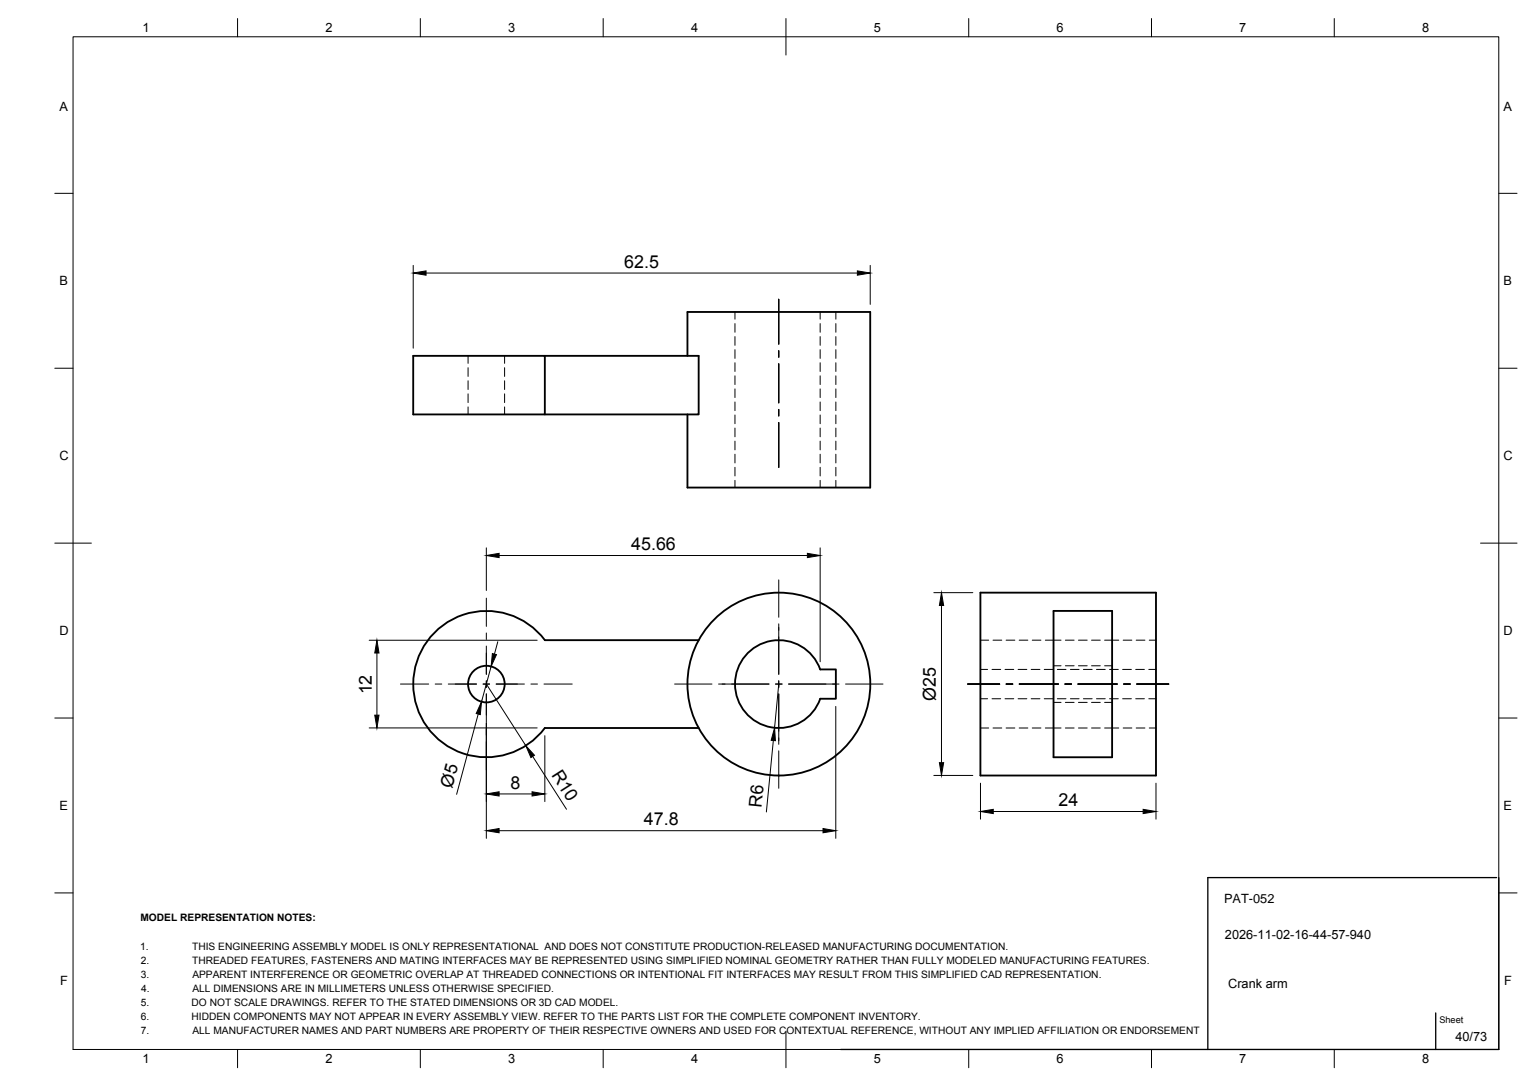
ISO-10303-21;
HEADER;
/* Generated by software containing ST-Developer
 * from STEP Tools, Inc. (www.steptools.com) 
 */

FILE_DESCRIPTION(
/* description */ ('Hand-crank gear train demonstrator'),
/* implementation_level */ '2;1');

FILE_NAME(
/* name */ 'Crank arm.step',
/* time_stamp */ '2026-10-28T03:22:13-07:00',
/* author */ (''),
/* organization */ (''),
/* preprocessor_version */ 'ST-DEVELOPER v20.2',
/* originating_system */ 'Autodesk Translation Framework v15.17.0.0',
/* authorisation */ '');

FILE_SCHEMA (('AUTOMOTIVE_DESIGN { 1 0 10303 214 3 1 1 }'));
ENDSEC;

DATA;
#10=MECHANICAL_DESIGN_GEOMETRIC_PRESENTATION_REPRESENTATION('',(#1236),#62758);
#1093=SHAPE_REPRESENTATION_RELATIONSHIP('SRR','None',#63068,#1157);
#1157=ADVANCED_BREP_SHAPE_REPRESENTATION('',(#1312),#62722);
#1236=STYLED_ITEM('',(#63455),#1312);
#1312=MANIFOLD_SOLID_BREP('Body1',#16419);
#1555=FACE_BOUND('',#3735,.T.);
#1556=FACE_BOUND('',#3739,.T.);
#1557=FACE_BOUND('',#3742,.T.);
#1558=FACE_BOUND('',#3745,.T.);
#1559=FACE_BOUND('',#3747,.T.);
#1906=PLANE('',#18042);
#1907=PLANE('',#18043);
#1908=PLANE('',#18044);
#1909=PLANE('',#18045);
#1910=PLANE('',#18053);
#1911=PLANE('',#18055);
#1912=PLANE('',#18056);
#1913=PLANE('',#18058);
#1914=PLANE('',#18061);
#2581=FACE_OUTER_BOUND('',#3730,.T.);
#2582=FACE_OUTER_BOUND('',#3731,.T.);
#2583=FACE_OUTER_BOUND('',#3732,.T.);
#2584=FACE_OUTER_BOUND('',#3733,.T.);
#2585=FACE_OUTER_BOUND('',#3734,.T.);
#2586=FACE_OUTER_BOUND('',#3736,.T.);
#2587=FACE_OUTER_BOUND('',#3737,.T.);
#2588=FACE_OUTER_BOUND('',#3738,.T.);
#2589=FACE_OUTER_BOUND('',#3740,.T.);
#2590=FACE_OUTER_BOUND('',#3741,.T.);
#2591=FACE_OUTER_BOUND('',#3743,.T.);
#2592=FACE_OUTER_BOUND('',#3744,.T.);
#2593=FACE_OUTER_BOUND('',#3746,.T.);
#3730=EDGE_LOOP('',(#12837,#12838,#12839,#12840));
#3731=EDGE_LOOP('',(#12841,#12842,#12843,#12844));
#3732=EDGE_LOOP('',(#12845,#12846,#12847,#12848));
#3733=EDGE_LOOP('',(#12849,#12850,#12851,#12852));
#3734=EDGE_LOOP('',(#12853));
#3735=EDGE_LOOP('',(#12854,#12855,#12856,#12857));
#3736=EDGE_LOOP('',(#12858,#12859,#12860,#12861));
#3737=EDGE_LOOP('',(#12862,#12863,#12864,#12865));
#3738=EDGE_LOOP('',(#12866,#12867,#12868,#12869));
#3739=EDGE_LOOP('',(#12870));
#3740=EDGE_LOOP('',(#12871,#12872,#12873,#12874));
#3741=EDGE_LOOP('',(#12875,#12876,#12877,#12878));
#3742=EDGE_LOOP('',(#12879));
#3743=EDGE_LOOP('',(#12880,#12881,#12882,#12883));
#3744=EDGE_LOOP('',(#12884,#12885,#12886,#12887));
#3745=EDGE_LOOP('',(#12888,#12889,#12890,#12891));
#3746=EDGE_LOOP('',(#12892));
#3747=EDGE_LOOP('',(#12893,#12894,#12895,#12896));
#4876=LINE('',#26186,#6008);
#4877=LINE('',#26191,#6009);
#4878=LINE('',#26193,#6010);
#4879=LINE('',#26195,#6011);
#4880=LINE('',#26196,#6012);
#4881=LINE('',#26199,#6013);
#4882=LINE('',#26201,#6014);
#4883=LINE('',#26202,#6015);
#4884=LINE('',#26205,#6016);
#4885=LINE('',#26207,#6017);
#4886=LINE('',#26208,#6018);
#4887=LINE('',#26218,#6019);
#4888=LINE('',#26222,#6020);
#4889=LINE('',#26226,#6021);
#4890=LINE('',#26229,#6022);
#4891=LINE('',#26232,#6023);
#4892=LINE('',#26233,#6024);
#4893=LINE('',#26236,#6025);
#4894=LINE('',#26239,#6026);
#4895=LINE('',#26242,#6027);
#6008=VECTOR('',#21187,0.25);
#6009=VECTOR('',#21192,1.);
#6010=VECTOR('',#21193,1.);
#6011=VECTOR('',#21194,1.);
#6012=VECTOR('',#21195,1.);
#6013=VECTOR('',#21198,1.);
#6014=VECTOR('',#21199,1.);
#6015=VECTOR('',#21200,1.);
#6016=VECTOR('',#21203,1.);
#6017=VECTOR('',#21204,1.);
#6018=VECTOR('',#21205,1.);
#6019=VECTOR('',#21218,1.);
#6020=VECTOR('',#21221,1.);
#6021=VECTOR('',#21226,1.);
#6022=VECTOR('',#21229,1.);
#6023=VECTOR('',#21232,1.);
#6024=VECTOR('',#21233,1.);
#6025=VECTOR('',#21236,1.);
#6026=VECTOR('',#21241,1.);
#6027=VECTOR('',#21244,1.25);
#6925=CIRCLE('',#18040,0.25);
#6926=CIRCLE('',#18041,0.25);
#6927=CIRCLE('',#18046,1.25);
#6928=CIRCLE('',#18047,0.6);
#6929=CIRCLE('',#18049,0.6);
#6930=CIRCLE('',#18051,1.);
#6931=CIRCLE('',#18052,1.);
#6932=CIRCLE('',#18054,1.25);
#6933=CIRCLE('',#18057,1.25);
#6934=CIRCLE('',#18060,1.25);
#7894=VERTEX_POINT('',#26183);
#7895=VERTEX_POINT('',#26185);
#7896=VERTEX_POINT('',#26189);
#7897=VERTEX_POINT('',#26190);
#7898=VERTEX_POINT('',#26192);
#7899=VERTEX_POINT('',#26194);
#7900=VERTEX_POINT('',#26198);
#7901=VERTEX_POINT('',#26200);
#7902=VERTEX_POINT('',#26204);
#7903=VERTEX_POINT('',#26206);
#7904=VERTEX_POINT('',#26210);
#7905=VERTEX_POINT('',#26216);
#7906=VERTEX_POINT('',#26217);
#7907=VERTEX_POINT('',#26219);
#7908=VERTEX_POINT('',#26221);
#7909=VERTEX_POINT('',#26225);
#7910=VERTEX_POINT('',#26227);
#7911=VERTEX_POINT('',#26231);
#7912=VERTEX_POINT('',#26235);
#7913=VERTEX_POINT('',#26241);
#9670=EDGE_CURVE('',#7894,#7894,#6925,.T.);
#9671=EDGE_CURVE('',#7894,#7895,#4876,.T.);
#9672=EDGE_CURVE('',#7895,#7895,#6926,.T.);
#9673=EDGE_CURVE('',#7896,#7897,#4877,.T.);
#9674=EDGE_CURVE('',#7896,#7898,#4878,.T.);
#9675=EDGE_CURVE('',#7899,#7898,#4879,.T.);
#9676=EDGE_CURVE('',#7897,#7899,#4880,.T.);
#9677=EDGE_CURVE('',#7900,#7896,#4881,.T.);
#9678=EDGE_CURVE('',#7900,#7901,#4882,.T.);
#9679=EDGE_CURVE('',#7898,#7901,#4883,.T.);
#9680=EDGE_CURVE('',#7902,#7900,#4884,.T.);
#9681=EDGE_CURVE('',#7903,#7902,#4885,.T.);
#9682=EDGE_CURVE('',#7901,#7903,#4886,.T.);
#9683=EDGE_CURVE('',#7904,#7904,#6927,.T.);
#9684=EDGE_CURVE('',#7903,#7899,#6928,.T.);
#9685=EDGE_CURVE('',#7902,#7897,#6929,.T.);
#9686=EDGE_CURVE('',#7905,#7906,#4887,.T.);
#9687=EDGE_CURVE('',#7907,#7905,#6930,.T.);
#9688=EDGE_CURVE('',#7908,#7907,#4888,.T.);
#9689=EDGE_CURVE('',#7908,#7906,#6931,.T.);
#9690=EDGE_CURVE('',#7908,#7909,#4889,.T.);
#9691=EDGE_CURVE('',#7910,#7909,#6932,.T.);
#9692=EDGE_CURVE('',#7910,#7906,#4890,.T.);
#9693=EDGE_CURVE('',#7911,#7907,#4891,.T.);
#9694=EDGE_CURVE('',#7909,#7911,#4892,.T.);
#9695=EDGE_CURVE('',#7905,#7912,#4893,.T.);
#9696=EDGE_CURVE('',#7911,#7912,#6933,.T.);
#9697=EDGE_CURVE('',#7912,#7910,#4894,.T.);
#9698=EDGE_CURVE('',#7904,#7913,#4895,.T.);
#9699=EDGE_CURVE('',#7913,#7913,#6934,.T.);
#12837=ORIENTED_EDGE('',*,*,#9670,.F.);
#12838=ORIENTED_EDGE('',*,*,#9671,.T.);
#12839=ORIENTED_EDGE('',*,*,#9672,.F.);
#12840=ORIENTED_EDGE('',*,*,#9671,.F.);
#12841=ORIENTED_EDGE('',*,*,#9673,.F.);
#12842=ORIENTED_EDGE('',*,*,#9674,.T.);
#12843=ORIENTED_EDGE('',*,*,#9675,.F.);
#12844=ORIENTED_EDGE('',*,*,#9676,.F.);
#12845=ORIENTED_EDGE('',*,*,#9677,.F.);
#12846=ORIENTED_EDGE('',*,*,#9678,.T.);
#12847=ORIENTED_EDGE('',*,*,#9679,.F.);
#12848=ORIENTED_EDGE('',*,*,#9674,.F.);
#12849=ORIENTED_EDGE('',*,*,#9680,.F.);
#12850=ORIENTED_EDGE('',*,*,#9681,.F.);
#12851=ORIENTED_EDGE('',*,*,#9682,.F.);
#12852=ORIENTED_EDGE('',*,*,#9678,.F.);
#12853=ORIENTED_EDGE('',*,*,#9683,.T.);
#12854=ORIENTED_EDGE('',*,*,#9675,.T.);
#12855=ORIENTED_EDGE('',*,*,#9679,.T.);
#12856=ORIENTED_EDGE('',*,*,#9682,.T.);
#12857=ORIENTED_EDGE('',*,*,#9684,.T.);
#12858=ORIENTED_EDGE('',*,*,#9676,.T.);
#12859=ORIENTED_EDGE('',*,*,#9684,.F.);
#12860=ORIENTED_EDGE('',*,*,#9681,.T.);
#12861=ORIENTED_EDGE('',*,*,#9685,.T.);
#12862=ORIENTED_EDGE('',*,*,#9686,.F.);
#12863=ORIENTED_EDGE('',*,*,#9687,.F.);
#12864=ORIENTED_EDGE('',*,*,#9688,.F.);
#12865=ORIENTED_EDGE('',*,*,#9689,.T.);
#12866=ORIENTED_EDGE('',*,*,#9689,.F.);
#12867=ORIENTED_EDGE('',*,*,#9690,.T.);
#12868=ORIENTED_EDGE('',*,*,#9691,.F.);
#12869=ORIENTED_EDGE('',*,*,#9692,.T.);
#12870=ORIENTED_EDGE('',*,*,#9670,.T.);
#12871=ORIENTED_EDGE('',*,*,#9688,.T.);
#12872=ORIENTED_EDGE('',*,*,#9693,.F.);
#12873=ORIENTED_EDGE('',*,*,#9694,.F.);
#12874=ORIENTED_EDGE('',*,*,#9690,.F.);
#12875=ORIENTED_EDGE('',*,*,#9695,.T.);
#12876=ORIENTED_EDGE('',*,*,#9696,.F.);
#12877=ORIENTED_EDGE('',*,*,#9693,.T.);
#12878=ORIENTED_EDGE('',*,*,#9687,.T.);
#12879=ORIENTED_EDGE('',*,*,#9672,.T.);
#12880=ORIENTED_EDGE('',*,*,#9686,.T.);
#12881=ORIENTED_EDGE('',*,*,#9692,.F.);
#12882=ORIENTED_EDGE('',*,*,#9697,.F.);
#12883=ORIENTED_EDGE('',*,*,#9695,.F.);
#12884=ORIENTED_EDGE('',*,*,#9683,.F.);
#12885=ORIENTED_EDGE('',*,*,#9698,.T.);
#12886=ORIENTED_EDGE('',*,*,#9699,.T.);
#12887=ORIENTED_EDGE('',*,*,#9698,.F.);
#12888=ORIENTED_EDGE('',*,*,#9697,.T.);
#12889=ORIENTED_EDGE('',*,*,#9691,.T.);
#12890=ORIENTED_EDGE('',*,*,#9694,.T.);
#12891=ORIENTED_EDGE('',*,*,#9696,.T.);
#12892=ORIENTED_EDGE('',*,*,#9699,.F.);
#12893=ORIENTED_EDGE('',*,*,#9673,.T.);
#12894=ORIENTED_EDGE('',*,*,#9685,.F.);
#12895=ORIENTED_EDGE('',*,*,#9680,.T.);
#12896=ORIENTED_EDGE('',*,*,#9677,.T.);
#15301=CYLINDRICAL_SURFACE('',#18039,0.25);
#15302=CYLINDRICAL_SURFACE('',#18048,0.6);
#15303=CYLINDRICAL_SURFACE('',#18050,1.);
#15304=CYLINDRICAL_SURFACE('',#18059,1.25);
#15891=ADVANCED_FACE('',(#2581),#15301,.F.);
#15892=ADVANCED_FACE('',(#2582),#1906,.F.);
#15893=ADVANCED_FACE('',(#2583),#1907,.F.);
#15894=ADVANCED_FACE('',(#2584),#1908,.F.);
#15895=ADVANCED_FACE('',(#2585,#1555),#1909,.T.);
#15896=ADVANCED_FACE('',(#2586),#15302,.F.);
#15897=ADVANCED_FACE('',(#2587),#15303,.T.);
#15898=ADVANCED_FACE('',(#2588,#1556),#1910,.F.);
#15899=ADVANCED_FACE('',(#2589),#1911,.T.);
#15900=ADVANCED_FACE('',(#2590,#1557),#1912,.T.);
#15901=ADVANCED_FACE('',(#2591),#1913,.T.);
#15902=ADVANCED_FACE('',(#2592,#1558),#15304,.T.);
#15903=ADVANCED_FACE('',(#2593,#1559),#1914,.F.);
#16419=CLOSED_SHELL('',(#15891,#15892,#15893,#15894,#15895,#15896,#15897,
#15898,#15899,#15900,#15901,#15902,#15903));
#18038=AXIS2_PLACEMENT_3D('',#26181,#21181,#21182);
#18039=AXIS2_PLACEMENT_3D('',#26182,#21183,#21184);
#18040=AXIS2_PLACEMENT_3D('',#26184,#21185,#21186);
#18041=AXIS2_PLACEMENT_3D('',#26187,#21188,#21189);
#18042=AXIS2_PLACEMENT_3D('',#26188,#21190,#21191);
#18043=AXIS2_PLACEMENT_3D('',#26197,#21196,#21197);
#18044=AXIS2_PLACEMENT_3D('',#26203,#21201,#21202);
#18045=AXIS2_PLACEMENT_3D('',#26209,#21206,#21207);
#18046=AXIS2_PLACEMENT_3D('',#26211,#21208,#21209);
#18047=AXIS2_PLACEMENT_3D('',#26212,#21210,#21211);
#18048=AXIS2_PLACEMENT_3D('',#26213,#21212,#21213);
#18049=AXIS2_PLACEMENT_3D('',#26214,#21214,#21215);
#18050=AXIS2_PLACEMENT_3D('',#26215,#21216,#21217);
#18051=AXIS2_PLACEMENT_3D('',#26220,#21219,#21220);
#18052=AXIS2_PLACEMENT_3D('',#26223,#21222,#21223);
#18053=AXIS2_PLACEMENT_3D('',#26224,#21224,#21225);
#18054=AXIS2_PLACEMENT_3D('',#26228,#21227,#21228);
#18055=AXIS2_PLACEMENT_3D('',#26230,#21230,#21231);
#18056=AXIS2_PLACEMENT_3D('',#26234,#21234,#21235);
#18057=AXIS2_PLACEMENT_3D('',#26237,#21237,#21238);
#18058=AXIS2_PLACEMENT_3D('',#26238,#21239,#21240);
#18059=AXIS2_PLACEMENT_3D('',#26240,#21242,#21243);
#18060=AXIS2_PLACEMENT_3D('',#26243,#21245,#21246);
#18061=AXIS2_PLACEMENT_3D('',#26244,#21247,#21248);
#21181=DIRECTION('axis',(0.,0.,1.));
#21182=DIRECTION('refdir',(1.,0.,0.));
#21183=DIRECTION('center_axis',(0.,1.,0.));
#21184=DIRECTION('ref_axis',(1.,0.,0.));
#21185=DIRECTION('center_axis',(0.,1.,0.));
#21186=DIRECTION('ref_axis',(1.,0.,0.));
#21187=DIRECTION('',(0.,1.,0.));
#21188=DIRECTION('center_axis',(0.,-1.,0.));
#21189=DIRECTION('ref_axis',(1.,0.,0.));
#21190=DIRECTION('center_axis',(-1.,0.,0.));
#21191=DIRECTION('ref_axis',(0.,0.,1.));
#21192=DIRECTION('',(0.,0.,1.));
#21193=DIRECTION('',(0.,1.,0.));
#21194=DIRECTION('',(0.,0.,-1.));
#21195=DIRECTION('',(0.,1.,0.));
#21196=DIRECTION('center_axis',(0.,0.,-1.));
#21197=DIRECTION('ref_axis',(-1.,0.,0.));
#21198=DIRECTION('',(-1.,0.,0.));
#21199=DIRECTION('',(0.,1.,0.));
#21200=DIRECTION('',(1.,0.,0.));
#21201=DIRECTION('center_axis',(1.,0.,0.));
#21202=DIRECTION('ref_axis',(0.,0.,-1.));
#21203=DIRECTION('',(0.,0.,-1.));
#21204=DIRECTION('',(0.,-1.,0.));
#21205=DIRECTION('',(0.,0.,1.));
#21206=DIRECTION('center_axis',(0.,1.,0.));
#21207=DIRECTION('ref_axis',(1.,0.,0.));
#21208=DIRECTION('center_axis',(0.,1.,0.));
#21209=DIRECTION('ref_axis',(1.,0.,0.));
#21210=DIRECTION('center_axis',(0.,-1.,0.));
#21211=DIRECTION('ref_axis',(1.,0.,0.));
#21212=DIRECTION('center_axis',(0.,1.,0.));
#21213=DIRECTION('ref_axis',(-1.83697019872103E-16,0.,1.));
#21214=DIRECTION('center_axis',(0.,-1.,0.));
#21215=DIRECTION('ref_axis',(1.,0.,0.));
#21216=DIRECTION('center_axis',(0.,1.,0.));
#21217=DIRECTION('ref_axis',(6.12323399573677E-17,0.,1.));
#21218=DIRECTION('',(0.,-1.,0.));
#21219=DIRECTION('center_axis',(0.,1.,0.));
#21220=DIRECTION('ref_axis',(1.,0.,0.));
#21221=DIRECTION('',(0.,1.,0.));
#21222=DIRECTION('center_axis',(0.,1.,0.));
#21223=DIRECTION('ref_axis',(1.,0.,0.));
#21224=DIRECTION('center_axis',(0.,1.,0.));
#21225=DIRECTION('ref_axis',(1.,0.,0.));
#21226=DIRECTION('',(0.,0.,-1.));
#21227=DIRECTION('center_axis',(0.,-1.,0.));
#21228=DIRECTION('ref_axis',(1.,0.,0.));
#21229=DIRECTION('',(0.,0.,1.));
#21230=DIRECTION('center_axis',(-1.,0.,0.));
#21231=DIRECTION('ref_axis',(0.,0.,1.));
#21232=DIRECTION('',(0.,0.,1.));
#21233=DIRECTION('',(0.,1.,0.));
#21234=DIRECTION('center_axis',(0.,1.,0.));
#21235=DIRECTION('ref_axis',(0.,0.,1.));
#21236=DIRECTION('',(0.,0.,-1.));
#21237=DIRECTION('center_axis',(0.,1.,0.));
#21238=DIRECTION('ref_axis',(1.,0.,0.));
#21239=DIRECTION('center_axis',(1.,0.,0.));
#21240=DIRECTION('ref_axis',(0.,0.,-1.));
#21241=DIRECTION('',(0.,-1.,0.));
#21242=DIRECTION('center_axis',(0.,1.,0.));
#21243=DIRECTION('ref_axis',(1.,0.,0.));
#21244=DIRECTION('',(0.,-1.,0.));
#21245=DIRECTION('center_axis',(0.,1.,0.));
#21246=DIRECTION('ref_axis',(1.,0.,0.));
#21247=DIRECTION('center_axis',(0.,1.,0.));
#21248=DIRECTION('ref_axis',(1.,0.,0.));
#26181=CARTESIAN_POINT('',(0.,0.,0.));
#26182=CARTESIAN_POINT('Origin',(0.,3.9,13.));
#26183=CARTESIAN_POINT('',(-0.25,4.,13.));
#26184=CARTESIAN_POINT('Origin',(0.,4.,13.));
#26185=CARTESIAN_POINT('',(-0.25,4.8,13.));
#26186=CARTESIAN_POINT('',(-0.25,3.9,13.));
#26187=CARTESIAN_POINT('Origin',(0.,4.8,13.));
#26188=CARTESIAN_POINT('Origin',(-0.2,3.3,8.22));
#26189=CARTESIAN_POINT('',(-0.2,3.4,8.22));
#26190=CARTESIAN_POINT('',(-0.2,3.4,8.43431457505076));
#26191=CARTESIAN_POINT('',(-0.2,3.4,8.61));
#26192=CARTESIAN_POINT('',(-0.2,5.8,8.22));
#26193=CARTESIAN_POINT('',(-0.2,3.3,8.22));
#26194=CARTESIAN_POINT('',(-0.2,5.8,8.43431457505076));
#26195=CARTESIAN_POINT('',(-0.2,5.8,8.61));
#26196=CARTESIAN_POINT('',(-0.2,3.4,8.43431457505076));
#26197=CARTESIAN_POINT('Origin',(0.2,3.3,8.22));
#26198=CARTESIAN_POINT('',(0.2,3.4,8.22));
#26199=CARTESIAN_POINT('',(0.1,3.4,8.22));
#26200=CARTESIAN_POINT('',(0.2,5.8,8.22));
#26201=CARTESIAN_POINT('',(0.2,3.3,8.22));
#26202=CARTESIAN_POINT('',(0.1,5.8,8.22));
#26203=CARTESIAN_POINT('Origin',(0.2,3.3,9.));
#26204=CARTESIAN_POINT('',(0.2,3.4,8.43431457505076));
#26205=CARTESIAN_POINT('',(0.2,3.4,9.));
#26206=CARTESIAN_POINT('',(0.2,5.8,8.43431457505076));
#26207=CARTESIAN_POINT('',(0.2,3.4,8.43431457505076));
#26208=CARTESIAN_POINT('',(0.2,5.8,9.));
#26209=CARTESIAN_POINT('Origin',(0.,5.8,9.));
#26210=CARTESIAN_POINT('',(-1.25,5.8,9.));
#26211=CARTESIAN_POINT('Origin',(0.,5.8,9.));
#26212=CARTESIAN_POINT('Origin',(0.,5.8,9.));
#26213=CARTESIAN_POINT('Origin',(0.,3.4,9.));
#26214=CARTESIAN_POINT('Origin',(0.,3.4,9.));
#26215=CARTESIAN_POINT('Origin',(0.,4.,13.));
#26216=CARTESIAN_POINT('',(0.6,4.8,12.2));
#26217=CARTESIAN_POINT('',(0.6,4.,12.2));
#26218=CARTESIAN_POINT('',(0.6,4.,12.2));
#26219=CARTESIAN_POINT('',(-0.6,4.8,12.2));
#26220=CARTESIAN_POINT('Origin',(0.,4.8,13.));
#26221=CARTESIAN_POINT('',(-0.6,4.,12.2));
#26222=CARTESIAN_POINT('',(-0.6,4.,12.2));
#26223=CARTESIAN_POINT('Origin',(0.,4.,13.));
#26224=CARTESIAN_POINT('Origin',(0.,4.,11.));
#26225=CARTESIAN_POINT('',(-0.6,4.,10.0965856099731));
#26226=CARTESIAN_POINT('',(-0.6,4.,13.));
#26227=CARTESIAN_POINT('',(0.6,4.,10.0965856099731));
#26228=CARTESIAN_POINT('Origin',(0.,4.,9.));
#26229=CARTESIAN_POINT('',(0.6,4.,9.));
#26230=CARTESIAN_POINT('Origin',(-0.6,4.,9.));
#26231=CARTESIAN_POINT('',(-0.6,4.8,10.0965856099731));
#26232=CARTESIAN_POINT('',(-0.6,4.8,13.));
#26233=CARTESIAN_POINT('',(-0.6,3.4,10.0965856099731));
#26234=CARTESIAN_POINT('Origin',(0.,4.8,11.));
#26235=CARTESIAN_POINT('',(0.6,4.8,10.0965856099731));
#26236=CARTESIAN_POINT('',(0.6,4.8,9.));
#26237=CARTESIAN_POINT('Origin',(0.,4.8,9.));
#26238=CARTESIAN_POINT('Origin',(0.6,4.,13.));
#26239=CARTESIAN_POINT('',(0.6,3.4,10.0965856099731));
#26240=CARTESIAN_POINT('Origin',(0.,3.4,9.));
#26241=CARTESIAN_POINT('',(-1.25,3.4,9.));
#26242=CARTESIAN_POINT('',(-1.25,3.4,9.));
#26243=CARTESIAN_POINT('Origin',(0.,3.4,9.));
#26244=CARTESIAN_POINT('Origin',(0.,3.4,9.));
#62648=UNCERTAINTY_MEASURE_WITH_UNIT(LENGTH_MEASURE(0.001),#62759,
'DISTANCE_ACCURACY_VALUE',
'Maximum model space distance between geometric entities at asserted c
onnectivities');
#62684=UNCERTAINTY_MEASURE_WITH_UNIT(LENGTH_MEASURE(0.001),#62759,
'DISTANCE_ACCURACY_VALUE',
'Maximum model space distance between geometric entities at asserted c
onnectivities');
#62722=(
GEOMETRIC_REPRESENTATION_CONTEXT(3)
GLOBAL_UNCERTAINTY_ASSIGNED_CONTEXT((#62648))
GLOBAL_UNIT_ASSIGNED_CONTEXT((#62759,#62761,#62762))
REPRESENTATION_CONTEXT('','3D')
);
#62758=(
GEOMETRIC_REPRESENTATION_CONTEXT(3)
GLOBAL_UNCERTAINTY_ASSIGNED_CONTEXT((#62684))
GLOBAL_UNIT_ASSIGNED_CONTEXT((#62759,#62761,#62762))
REPRESENTATION_CONTEXT('','3D')
);
#62759=(
LENGTH_UNIT()
NAMED_UNIT(*)
SI_UNIT(.CENTI.,.METRE.)
);
#62761=(
NAMED_UNIT(*)
PLANE_ANGLE_UNIT()
SI_UNIT($,.RADIAN.)
);
#62762=(
NAMED_UNIT(*)
SI_UNIT($,.STERADIAN.)
SOLID_ANGLE_UNIT()
);
#62800=SHAPE_DEFINITION_REPRESENTATION(#62883,#63068);
#62883=PRODUCT_DEFINITION_SHAPE('',$,#63142);
#63068=SHAPE_REPRESENTATION('',(#18038),#62722);
#63104=PRODUCT_DEFINITION_CONTEXT('part definition',#63325,'design');
#63142=PRODUCT_DEFINITION('Crank arm','Crank arm',#63215,#63104);
#63215=PRODUCT_DEFINITION_FORMATION('',$,#63364);
#63325=APPLICATION_CONTEXT(
'Core Data for Automotive Mechanical Design Process');
#63326=PRODUCT_CONTEXT('part definition',#63325,'mechanical');
#63364=PRODUCT('Crank arm','Crank arm','Crank arm',(#63326));
#63449=COLOUR_RGB('Sky Blue',0.24,0.69,0.87);
#63450=FILL_AREA_STYLE_COLOUR('',#63449);
#63451=FILL_AREA_STYLE('',(#63450));
#63452=SURFACE_STYLE_FILL_AREA(#63451);
#63453=SURFACE_SIDE_STYLE('',(#63452));
#63454=SURFACE_STYLE_USAGE(.BOTH.,#63453);
#63455=PRESENTATION_STYLE_ASSIGNMENT((#63454));
ENDSEC;
END-ISO-10303-21;
